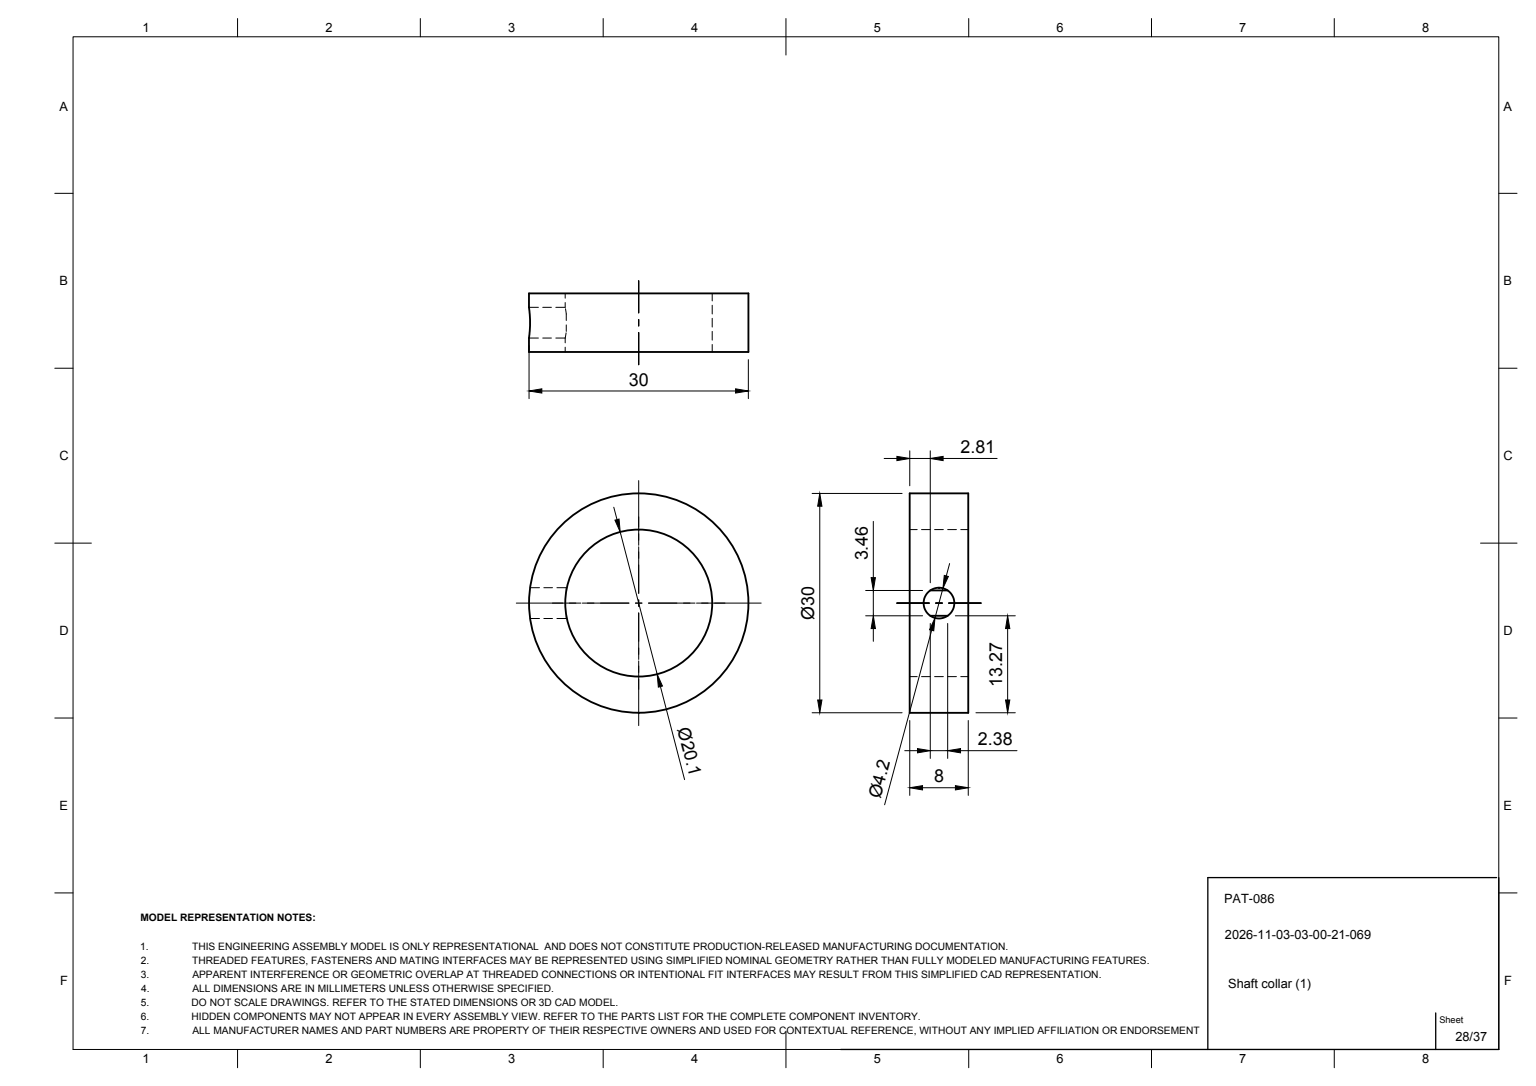
ISO-10303-21;
HEADER;
/* Generated by software containing ST-Developer
 * from STEP Tools, Inc. (www.steptools.com) 
 */

FILE_DESCRIPTION(
/* description */ ('Ratchet and pawl hand winch drum'),
/* implementation_level */ '2;1');

FILE_NAME(
/* name */ 'Shaft collar (1).step',
/* time_stamp */ '2026-10-27T12:42:58-07:00',
/* author */ (''),
/* organization */ (''),
/* preprocessor_version */ 'ST-DEVELOPER v20.2',
/* originating_system */ 'Autodesk Translation Framework v15.17.0.0',
/* authorisation */ '');

FILE_SCHEMA (('AUTOMOTIVE_DESIGN { 1 0 10303 214 3 1 1 }'));
ENDSEC;

DATA;
#10=MECHANICAL_DESIGN_GEOMETRIC_PRESENTATION_REPRESENTATION('',(#412),#11801);
#301=B_SPLINE_CURVE_WITH_KNOTS('',3,(#10693,#10694,#10695,#10696,#10697,
#10698,#10699,#10700,#10701,#10702,#10703,#10704,#10705,#10706),
 .UNSPECIFIED.,.F.,.F.,(4,2,2,2,2,2,4),(0.756005737987024,0.793568827564645,
0.8729225200542,0.952276212543755,1.03162990503331,1.11098359752287,1.14854668710049),
 .UNSPECIFIED.);
#302=B_SPLINE_CURVE_WITH_KNOTS('',3,(#10712,#10713,#10714,#10715,#10716,
#10717,#10718,#10719,#10720,#10721,#10722,#10723,#10724,#10725,#10726,#10727,
#10728,#10729),.UNSPECIFIED.,.F.,.F.,(4,2,2,2,2,2,2,2,4),(0.,0.0792165807733624,
0.158433161546725,0.23764869707457,0.316864232602414,0.396079768130259,
0.475295303658103,0.554511884431466,0.633728465204828),.UNSPECIFIED.);
#303=B_SPLINE_CURVE_WITH_KNOTS('',3,(#10730,#10731,#10732,#10733,#10734,
#10735,#10736,#10737,#10738,#10739,#10740,#10741,#10742,#10743,#10744,#10745,
#10746,#10747),.UNSPECIFIED.,.F.,.F.,(4,2,2,2,2,2,2,2,4),(0.633728465204828,
0.712945045978191,0.792161626751553,0.871377162279398,0.950592697807242,
1.02980823333509,1.10902376886293,1.18824034963629,1.26745693040966),
 .UNSPECIFIED.);
#304=B_SPLINE_CURVE_WITH_KNOTS('',3,(#10750,#10751,#10752,#10753,#10754,
#10755,#10756,#10757,#10758,#10759,#10760,#10761,#10762,#10763),
 .UNSPECIFIED.,.F.,.F.,(4,2,2,2,2,2,4),(0.121154929624523,0.158718019202141,
0.238071711691696,0.317425404181252,0.396779096670807,0.476132789160362,
0.51369587873798),.UNSPECIFIED.);
#343=SHAPE_REPRESENTATION_RELATIONSHIP('SRR','None',#11971,#377);
#377=ADVANCED_BREP_SHAPE_REPRESENTATION('',(#445),#11788);
#412=STYLED_ITEM('',(#12213),#445);
#445=MANIFOLD_SOLID_BREP('Body1',#6291);
#568=FACE_BOUND('',#1525,.T.);
#569=FACE_BOUND('',#1527,.T.);
#570=FACE_BOUND('',#1529,.T.);
#571=FACE_BOUND('',#1531,.T.);
#732=PLANE('',#7072);
#733=PLANE('',#7077);
#734=PLANE('',#7084);
#735=PLANE('',#7085);
#1053=FACE_OUTER_BOUND('',#1521,.T.);
#1054=FACE_OUTER_BOUND('',#1522,.T.);
#1055=FACE_OUTER_BOUND('',#1523,.T.);
#1056=FACE_OUTER_BOUND('',#1524,.T.);
#1057=FACE_OUTER_BOUND('',#1526,.T.);
#1058=FACE_OUTER_BOUND('',#1528,.T.);
#1059=FACE_OUTER_BOUND('',#1530,.T.);
#1521=EDGE_LOOP('',(#5139,#5140));
#1522=EDGE_LOOP('',(#5141,#5142,#5143,#5144,#5145,#5146,#5147,#5148,#5149));
#1523=EDGE_LOOP('',(#5150,#5151,#5152));
#1524=EDGE_LOOP('',(#5153,#5154,#5155,#5156));
#1525=EDGE_LOOP('',(#5157,#5158,#5159,#5160));
#1526=EDGE_LOOP('',(#5161,#5162,#5163,#5164));
#1527=EDGE_LOOP('',(#5165,#5166));
#1528=EDGE_LOOP('',(#5167));
#1529=EDGE_LOOP('',(#5168));
#1530=EDGE_LOOP('',(#5169));
#1531=EDGE_LOOP('',(#5170));
#1964=LINE('',#10689,#2475);
#1965=LINE('',#10710,#2476);
#1966=LINE('',#10765,#2477);
#1967=LINE('',#10770,#2478);
#1968=LINE('',#10776,#2479);
#2475=VECTOR('',#8413,1.);
#2476=VECTOR('',#8420,0.21);
#2477=VECTOR('',#8425,1.);
#2478=VECTOR('',#8430,1.005);
#2479=VECTOR('',#8437,1.5);
#2870=CIRCLE('',#7073,0.21);
#2871=CIRCLE('',#7075,0.21);
#2872=CIRCLE('',#7076,0.21);
#2873=CIRCLE('',#7079,1.005);
#2874=CIRCLE('',#7080,1.005);
#2875=CIRCLE('',#7082,1.5);
#2876=CIRCLE('',#7083,1.5);
#3245=VERTEX_POINT('',#10687);
#3246=VERTEX_POINT('',#10688);
#3247=VERTEX_POINT('',#10692);
#3248=VERTEX_POINT('',#10707);
#3249=VERTEX_POINT('',#10709);
#3250=VERTEX_POINT('',#10711);
#3251=VERTEX_POINT('',#10748);
#3252=VERTEX_POINT('',#10767);
#3253=VERTEX_POINT('',#10769);
#3254=VERTEX_POINT('',#10773);
#3255=VERTEX_POINT('',#10775);
#3913=EDGE_CURVE('',#3245,#3246,#1964,.T.);
#3914=EDGE_CURVE('',#3245,#3246,#2870,.T.);
#3915=EDGE_CURVE('',#3247,#3245,#301,.T.);
#3916=EDGE_CURVE('',#3248,#3247,#2871,.T.);
#3917=EDGE_CURVE('',#3248,#3249,#1965,.T.);
#3918=EDGE_CURVE('',#3250,#3249,#302,.T.);
#3919=EDGE_CURVE('',#3249,#3250,#303,.T.);
#3920=EDGE_CURVE('',#3251,#3248,#2872,.T.);
#3921=EDGE_CURVE('',#3246,#3251,#304,.T.);
#3922=EDGE_CURVE('',#3251,#3247,#1966,.T.);
#3923=EDGE_CURVE('',#3252,#3252,#2873,.T.);
#3924=EDGE_CURVE('',#3252,#3253,#1967,.T.);
#3925=EDGE_CURVE('',#3253,#3253,#2874,.T.);
#3926=EDGE_CURVE('',#3254,#3254,#2875,.T.);
#3927=EDGE_CURVE('',#3254,#3255,#1968,.T.);
#3928=EDGE_CURVE('',#3255,#3255,#2876,.T.);
#5139=ORIENTED_EDGE('',*,*,#3913,.F.);
#5140=ORIENTED_EDGE('',*,*,#3914,.T.);
#5141=ORIENTED_EDGE('',*,*,#3915,.F.);
#5142=ORIENTED_EDGE('',*,*,#3916,.F.);
#5143=ORIENTED_EDGE('',*,*,#3917,.T.);
#5144=ORIENTED_EDGE('',*,*,#3918,.F.);
#5145=ORIENTED_EDGE('',*,*,#3919,.F.);
#5146=ORIENTED_EDGE('',*,*,#3917,.F.);
#5147=ORIENTED_EDGE('',*,*,#3920,.F.);
#5148=ORIENTED_EDGE('',*,*,#3921,.F.);
#5149=ORIENTED_EDGE('',*,*,#3914,.F.);
#5150=ORIENTED_EDGE('',*,*,#3922,.F.);
#5151=ORIENTED_EDGE('',*,*,#3920,.T.);
#5152=ORIENTED_EDGE('',*,*,#3916,.T.);
#5153=ORIENTED_EDGE('',*,*,#3923,.F.);
#5154=ORIENTED_EDGE('',*,*,#3924,.T.);
#5155=ORIENTED_EDGE('',*,*,#3925,.T.);
#5156=ORIENTED_EDGE('',*,*,#3924,.F.);
#5157=ORIENTED_EDGE('',*,*,#3921,.T.);
#5158=ORIENTED_EDGE('',*,*,#3922,.T.);
#5159=ORIENTED_EDGE('',*,*,#3915,.T.);
#5160=ORIENTED_EDGE('',*,*,#3913,.T.);
#5161=ORIENTED_EDGE('',*,*,#3926,.F.);
#5162=ORIENTED_EDGE('',*,*,#3927,.T.);
#5163=ORIENTED_EDGE('',*,*,#3928,.T.);
#5164=ORIENTED_EDGE('',*,*,#3927,.F.);
#5165=ORIENTED_EDGE('',*,*,#3918,.T.);
#5166=ORIENTED_EDGE('',*,*,#3919,.T.);
#5167=ORIENTED_EDGE('',*,*,#3926,.T.);
#5168=ORIENTED_EDGE('',*,*,#3923,.T.);
#5169=ORIENTED_EDGE('',*,*,#3928,.F.);
#5170=ORIENTED_EDGE('',*,*,#3925,.F.);
#5881=CYLINDRICAL_SURFACE('',#7074,0.21);
#5882=CYLINDRICAL_SURFACE('',#7078,1.005);
#5883=CYLINDRICAL_SURFACE('',#7081,1.5);
#6123=ADVANCED_FACE('',(#1053),#732,.T.);
#6124=ADVANCED_FACE('',(#1054),#5881,.F.);
#6125=ADVANCED_FACE('',(#1055),#733,.T.);
#6126=ADVANCED_FACE('',(#1056,#568),#5882,.F.);
#6127=ADVANCED_FACE('',(#1057,#569),#5883,.T.);
#6128=ADVANCED_FACE('',(#1058,#570),#734,.T.);
#6129=ADVANCED_FACE('',(#1059,#571),#735,.F.);
#6291=CLOSED_SHELL('',(#6123,#6124,#6125,#6126,#6127,#6128,#6129));
#7071=AXIS2_PLACEMENT_3D('',#10685,#8409,#8410);
#7072=AXIS2_PLACEMENT_3D('',#10686,#8411,#8412);
#7073=AXIS2_PLACEMENT_3D('',#10690,#8414,#8415);
#7074=AXIS2_PLACEMENT_3D('',#10691,#8416,#8417);
#7075=AXIS2_PLACEMENT_3D('',#10708,#8418,#8419);
#7076=AXIS2_PLACEMENT_3D('',#10749,#8421,#8422);
#7077=AXIS2_PLACEMENT_3D('',#10764,#8423,#8424);
#7078=AXIS2_PLACEMENT_3D('',#10766,#8426,#8427);
#7079=AXIS2_PLACEMENT_3D('',#10768,#8428,#8429);
#7080=AXIS2_PLACEMENT_3D('',#10771,#8431,#8432);
#7081=AXIS2_PLACEMENT_3D('',#10772,#8433,#8434);
#7082=AXIS2_PLACEMENT_3D('',#10774,#8435,#8436);
#7083=AXIS2_PLACEMENT_3D('',#10777,#8438,#8439);
#7084=AXIS2_PLACEMENT_3D('',#10778,#8440,#8441);
#7085=AXIS2_PLACEMENT_3D('',#10779,#8442,#8443);
#8409=DIRECTION('axis',(0.,0.,1.));
#8410=DIRECTION('refdir',(1.,0.,0.));
#8411=DIRECTION('center_axis',(0.,0.,1.));
#8412=DIRECTION('ref_axis',(1.,0.,0.));
#8413=DIRECTION('',(0.,1.,0.));
#8414=DIRECTION('center_axis',(0.,0.,1.));
#8415=DIRECTION('ref_axis',(1.,0.,0.));
#8416=DIRECTION('center_axis',(0.,0.,1.));
#8417=DIRECTION('ref_axis',(1.,0.,0.));
#8418=DIRECTION('center_axis',(0.,0.,1.));
#8419=DIRECTION('ref_axis',(1.,0.,0.));
#8420=DIRECTION('',(0.,0.,1.));
#8421=DIRECTION('center_axis',(0.,0.,1.));
#8422=DIRECTION('ref_axis',(1.,0.,0.));
#8423=DIRECTION('center_axis',(0.,0.,1.));
#8424=DIRECTION('ref_axis',(1.,0.,0.));
#8425=DIRECTION('',(0.,-1.,0.));
#8426=DIRECTION('center_axis',(0.,1.,0.));
#8427=DIRECTION('ref_axis',(1.,0.,0.));
#8428=DIRECTION('center_axis',(0.,-1.,0.));
#8429=DIRECTION('ref_axis',(1.,0.,0.));
#8430=DIRECTION('',(0.,-1.,0.));
#8431=DIRECTION('center_axis',(0.,-1.,0.));
#8432=DIRECTION('ref_axis',(1.,0.,0.));
#8433=DIRECTION('center_axis',(0.,1.,0.));
#8434=DIRECTION('ref_axis',(1.,0.,0.));
#8435=DIRECTION('center_axis',(0.,1.,0.));
#8436=DIRECTION('ref_axis',(1.,0.,0.));
#8437=DIRECTION('',(0.,-1.,0.));
#8438=DIRECTION('center_axis',(0.,1.,0.));
#8439=DIRECTION('ref_axis',(1.,0.,0.));
#8440=DIRECTION('center_axis',(0.,1.,0.));
#8441=DIRECTION('ref_axis',(1.,0.,0.));
#8442=DIRECTION('center_axis',(0.,1.,0.));
#8443=DIRECTION('ref_axis',(1.,0.,0.));
#10685=CARTESIAN_POINT('',(0.,0.,0.));
#10686=CARTESIAN_POINT('Origin',(0.,18.85,7.52));
#10687=CARTESIAN_POINT('',(0.172988438920056,18.7309411910021,7.52));
#10688=CARTESIAN_POINT('',(0.172988438920056,18.9690588089979,7.52));
#10689=CARTESIAN_POINT('',(0.172988438920056,18.45,7.52));
#10690=CARTESIAN_POINT('Origin',(0.,18.85,7.52));
#10691=CARTESIAN_POINT('Origin',(0.,18.85,7.52));
#10692=CARTESIAN_POINT('',(-0.172988438920056,18.7309411910021,7.52));
#10693=CARTESIAN_POINT('Ctrl Pts',(-0.172988438920055,18.7309411910021,
7.52));
#10694=CARTESIAN_POINT('Ctrl Pts',(-0.165594865311313,18.7201985776047,
7.52129192197638));
#10695=CARTESIAN_POINT('Ctrl Pts',(-0.157297138725605,18.7103122906273,
7.52265394943905));
#10696=CARTESIAN_POINT('Ctrl Pts',(-0.129892073845076,18.6829072257467,
7.5267480843909));
#10697=CARTESIAN_POINT('Ctrl Pts',(-0.106330167759285,18.6667579436671,
7.52969589327637));
#10698=CARTESIAN_POINT('Ctrl Pts',(-0.0546129046324106,18.6453022060351,
7.53385029472357));
#10699=CARTESIAN_POINT('Ctrl Pts',(-0.0264512308298518,18.64,7.535));
#10700=CARTESIAN_POINT('Ctrl Pts',(0.0264512308298517,18.64,7.535));
#10701=CARTESIAN_POINT('Ctrl Pts',(0.0546129046324104,18.6453022060351,
7.53385029472357));
#10702=CARTESIAN_POINT('Ctrl Pts',(0.106330167759284,18.6667579436671,7.52969589327638));
#10703=CARTESIAN_POINT('Ctrl Pts',(0.129892073845076,18.6829072257467,7.5267480843909));
#10704=CARTESIAN_POINT('Ctrl Pts',(0.157297138725605,18.7103122906273,7.52265394943905));
#10705=CARTESIAN_POINT('Ctrl Pts',(0.165594865311314,18.7201985776047,7.52129192197638));
#10706=CARTESIAN_POINT('Ctrl Pts',(0.172988438920056,18.7309411910021,7.52));
#10707=CARTESIAN_POINT('',(-0.21,18.85,7.52));
#10708=CARTESIAN_POINT('Origin',(0.,18.85,7.52));
#10709=CARTESIAN_POINT('',(-0.21,18.85,8.01522725533839));
#10710=CARTESIAN_POINT('',(-0.21,18.85,7.52));
#10711=CARTESIAN_POINT('',(0.21,18.85,8.01522725533839));
#10712=CARTESIAN_POINT('Ctrl Pts',(0.21,18.85,8.01522725533839));
#10713=CARTESIAN_POINT('Ctrl Pts',(0.21,18.8235944730755,8.01522725533839));
#10714=CARTESIAN_POINT('Ctrl Pts',(0.204715737269595,18.7954529259093,8.01600415954412));
#10715=CARTESIAN_POINT('Ctrl Pts',(0.18327376303633,18.7437237310949,8.01880073282317));
#10716=CARTESIAN_POINT('Ctrl Pts',(0.167117923970393,18.720133075872,8.02077897157582));
#10717=CARTESIAN_POINT('Ctrl Pts',(0.129867169887369,18.682882321789,8.02448481141327));
#10718=CARTESIAN_POINT('Ctrl Pts',(0.106276408305767,18.6667262899986,8.02645455657129));
#10719=CARTESIAN_POINT('Ctrl Pts',(0.0545468514059018,18.6452841751738,
8.02923165515645));
#10720=CARTESIAN_POINT('Ctrl Pts',(0.0264051785092816,18.64,8.03));
#10721=CARTESIAN_POINT('Ctrl Pts',(-0.0264051785092815,18.64,8.03));
#10722=CARTESIAN_POINT('Ctrl Pts',(-0.0545468514059018,18.6452841751738,
8.02923165515645));
#10723=CARTESIAN_POINT('Ctrl Pts',(-0.106276408305767,18.6667262899986,
8.02645455657129));
#10724=CARTESIAN_POINT('Ctrl Pts',(-0.129867169887368,18.682882321789,8.02448481141327));
#10725=CARTESIAN_POINT('Ctrl Pts',(-0.167117923970393,18.720133075872,8.02077897157582));
#10726=CARTESIAN_POINT('Ctrl Pts',(-0.18327376303633,18.7437237310949,8.01880073282317));
#10727=CARTESIAN_POINT('Ctrl Pts',(-0.204715737269595,18.7954529259093,
8.01600415954412));
#10728=CARTESIAN_POINT('Ctrl Pts',(-0.21,18.8235944730755,8.01522725533839));
#10729=CARTESIAN_POINT('Ctrl Pts',(-0.21,18.85,8.01522725533839));
#10730=CARTESIAN_POINT('Ctrl Pts',(-0.21,18.85,8.01522725533839));
#10731=CARTESIAN_POINT('Ctrl Pts',(-0.21,18.8764055269245,8.01522725533839));
#10732=CARTESIAN_POINT('Ctrl Pts',(-0.204715737269595,18.9045470740907,
8.01600415954412));
#10733=CARTESIAN_POINT('Ctrl Pts',(-0.18327376303633,18.9562762689051,8.01880073282317));
#10734=CARTESIAN_POINT('Ctrl Pts',(-0.167117923970393,18.979866924128,8.02077897157582));
#10735=CARTESIAN_POINT('Ctrl Pts',(-0.129867169887369,19.017117678211,8.02448481141327));
#10736=CARTESIAN_POINT('Ctrl Pts',(-0.106276408305767,19.0332737100014,
8.02645455657129));
#10737=CARTESIAN_POINT('Ctrl Pts',(-0.0545468514059018,19.0547158248262,
8.02923165515645));
#10738=CARTESIAN_POINT('Ctrl Pts',(-0.0264051785092816,19.06,8.03));
#10739=CARTESIAN_POINT('Ctrl Pts',(0.0264051785092815,19.06,8.03));
#10740=CARTESIAN_POINT('Ctrl Pts',(0.0545468514059019,19.0547158248262,
8.02923165515645));
#10741=CARTESIAN_POINT('Ctrl Pts',(0.106276408305767,19.0332737100014,8.02645455657129));
#10742=CARTESIAN_POINT('Ctrl Pts',(0.129867169887368,19.017117678211,8.02448481141327));
#10743=CARTESIAN_POINT('Ctrl Pts',(0.167117923970393,18.979866924128,8.02077897157582));
#10744=CARTESIAN_POINT('Ctrl Pts',(0.18327376303633,18.9562762689051,8.01880073282317));
#10745=CARTESIAN_POINT('Ctrl Pts',(0.204715737269595,18.9045470740907,8.01600415954412));
#10746=CARTESIAN_POINT('Ctrl Pts',(0.21,18.8764055269245,8.01522725533839));
#10747=CARTESIAN_POINT('Ctrl Pts',(0.21,18.85,8.01522725533839));
#10748=CARTESIAN_POINT('',(-0.172988438920056,18.9690588089979,7.52));
#10749=CARTESIAN_POINT('Origin',(0.,18.85,7.52));
#10750=CARTESIAN_POINT('Ctrl Pts',(0.172988438920053,18.9690588089979,7.52));
#10751=CARTESIAN_POINT('Ctrl Pts',(0.165594865311312,18.9798014223953,7.52129192197638));
#10752=CARTESIAN_POINT('Ctrl Pts',(0.157297138725604,18.9896877093727,7.52265394943905));
#10753=CARTESIAN_POINT('Ctrl Pts',(0.129892073845076,19.0170927742533,7.5267480843909));
#10754=CARTESIAN_POINT('Ctrl Pts',(0.106330167759284,19.033242056333,7.52969589327638));
#10755=CARTESIAN_POINT('Ctrl Pts',(0.0546129046324105,19.0546977939649,
7.53385029472357));
#10756=CARTESIAN_POINT('Ctrl Pts',(0.0264512308298518,19.06,7.535));
#10757=CARTESIAN_POINT('Ctrl Pts',(-0.0264512308298517,19.06,7.535));
#10758=CARTESIAN_POINT('Ctrl Pts',(-0.0546129046324105,19.0546977939649,
7.53385029472357));
#10759=CARTESIAN_POINT('Ctrl Pts',(-0.106330167759284,19.033242056333,7.52969589327638));
#10760=CARTESIAN_POINT('Ctrl Pts',(-0.129892073845076,19.0170927742533,
7.5267480843909));
#10761=CARTESIAN_POINT('Ctrl Pts',(-0.157297138725604,18.9896877093727,
7.52265394943905));
#10762=CARTESIAN_POINT('Ctrl Pts',(-0.165594865311312,18.9798014223953,
7.52129192197638));
#10763=CARTESIAN_POINT('Ctrl Pts',(-0.172988438920053,18.9690588089979,
7.52));
#10764=CARTESIAN_POINT('Origin',(0.,18.85,7.52));
#10765=CARTESIAN_POINT('',(-0.172988438920056,18.45,7.52));
#10766=CARTESIAN_POINT('Origin',(0.,18.45,6.53));
#10767=CARTESIAN_POINT('',(-1.005,19.25,6.53));
#10768=CARTESIAN_POINT('Origin',(0.,19.25,6.53));
#10769=CARTESIAN_POINT('',(-1.005,18.45,6.53));
#10770=CARTESIAN_POINT('',(-1.005,18.45,6.53));
#10771=CARTESIAN_POINT('Origin',(0.,18.45,6.53));
#10772=CARTESIAN_POINT('Origin',(0.,18.45,6.53));
#10773=CARTESIAN_POINT('',(-1.5,19.25,6.53));
#10774=CARTESIAN_POINT('Origin',(0.,19.25,6.53));
#10775=CARTESIAN_POINT('',(-1.5,18.45,6.53));
#10776=CARTESIAN_POINT('',(-1.5,18.45,6.53));
#10777=CARTESIAN_POINT('Origin',(0.,18.45,6.53));
#10778=CARTESIAN_POINT('Origin',(0.,19.25,6.53));
#10779=CARTESIAN_POINT('Origin',(0.,18.45,6.53));
#11748=UNCERTAINTY_MEASURE_WITH_UNIT(LENGTH_MEASURE(0.001),#11802,
'DISTANCE_ACCURACY_VALUE',
'Maximum model space distance between geometric entities at asserted c
onnectivities');
#11761=UNCERTAINTY_MEASURE_WITH_UNIT(LENGTH_MEASURE(0.001),#11802,
'DISTANCE_ACCURACY_VALUE',
'Maximum model space distance between geometric entities at asserted c
onnectivities');
#11788=(
GEOMETRIC_REPRESENTATION_CONTEXT(3)
GLOBAL_UNCERTAINTY_ASSIGNED_CONTEXT((#11748))
GLOBAL_UNIT_ASSIGNED_CONTEXT((#11802,#11804,#11805))
REPRESENTATION_CONTEXT('','3D')
);
#11801=(
GEOMETRIC_REPRESENTATION_CONTEXT(3)
GLOBAL_UNCERTAINTY_ASSIGNED_CONTEXT((#11761))
GLOBAL_UNIT_ASSIGNED_CONTEXT((#11802,#11804,#11805))
REPRESENTATION_CONTEXT('','3D')
);
#11802=(
LENGTH_UNIT()
NAMED_UNIT(*)
SI_UNIT(.CENTI.,.METRE.)
);
#11804=(
NAMED_UNIT(*)
PLANE_ANGLE_UNIT()
SI_UNIT($,.RADIAN.)
);
#11805=(
NAMED_UNIT(*)
SI_UNIT($,.STERADIAN.)
SOLID_ANGLE_UNIT()
);
#11832=SHAPE_DEFINITION_REPRESENTATION(#11873,#11971);
#11873=PRODUCT_DEFINITION_SHAPE('',$,#12011);
#11971=SHAPE_REPRESENTATION('',(#7071),#11788);
#11984=PRODUCT_DEFINITION_CONTEXT('part definition',#12103,'design');
#12011=PRODUCT_DEFINITION('Shaft collar (1)','Shaft collar (1)',#12050,#11984);
#12050=PRODUCT_DEFINITION_FORMATION('',$,#12131);
#12103=APPLICATION_CONTEXT(
'Core Data for Automotive Mechanical Design Process');
#12104=PRODUCT_CONTEXT('part definition',#12103,'mechanical');
#12131=PRODUCT('Shaft collar (1)','Shaft collar (1)','Shaft collar (1)',(#12104));
#12207=COLOUR_RGB('Grey',0.48,0.52,0.57);
#12208=FILL_AREA_STYLE_COLOUR('',#12207);
#12209=FILL_AREA_STYLE('',(#12208));
#12210=SURFACE_STYLE_FILL_AREA(#12209);
#12211=SURFACE_SIDE_STYLE('',(#12210));
#12212=SURFACE_STYLE_USAGE(.BOTH.,#12211);
#12213=PRESENTATION_STYLE_ASSIGNMENT((#12212));
ENDSEC;
END-ISO-10303-21;
